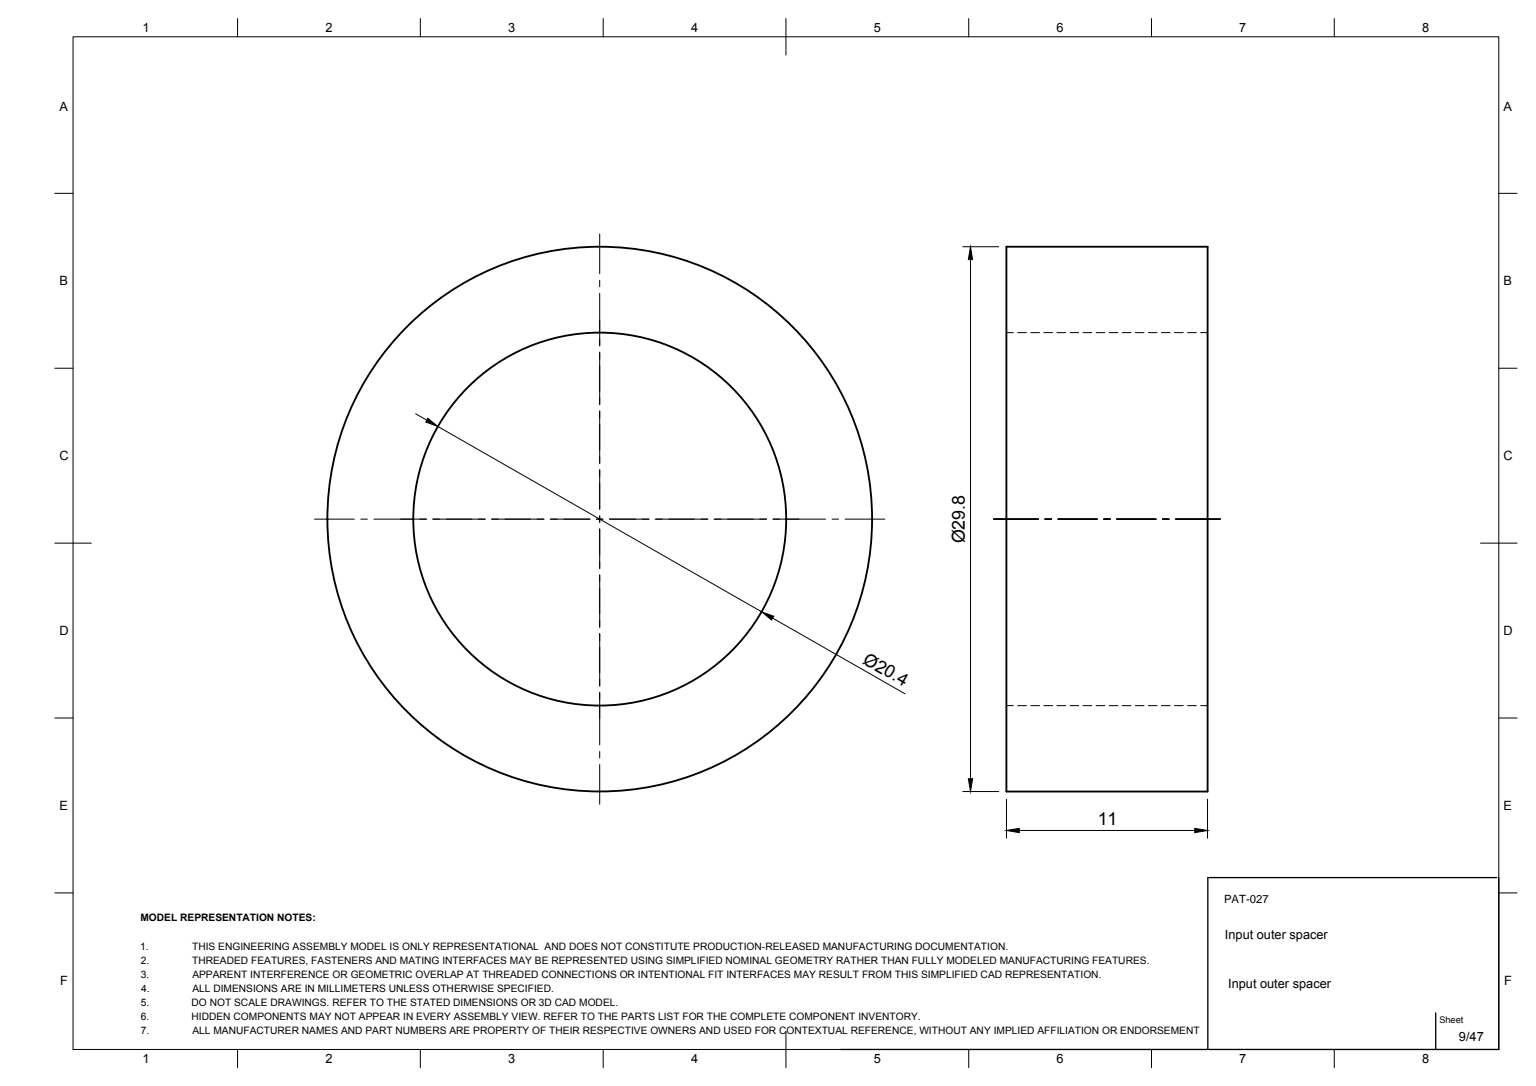
ISO-10303-21;
HEADER;
/* Generated by software containing ST-Developer
 * from STEP Tools, Inc. (www.steptools.com) 
 */

FILE_DESCRIPTION(
/* description */ ('Crank-driven oscillating fan base (mechanism only)'),

/* implementation_level */ '2;1');

FILE_NAME(
/* name */ 'Input outer spacer.step',
/* time_stamp */ '2026-10-28T03:25:00-07:00',
/* author */ (''),
/* organization */ (''),
/* preprocessor_version */ 'ST-DEVELOPER v20.2',
/* originating_system */ 'Autodesk Translation Framework v15.17.0.0',
/* authorisation */ '');

FILE_SCHEMA (('AUTOMOTIVE_DESIGN { 1 0 10303 214 3 1 1 }'));
ENDSEC;

DATA;
#10=MECHANICAL_DESIGN_GEOMETRIC_PRESENTATION_REPRESENTATION('',(#441),#11916);
#361=SHAPE_REPRESENTATION_RELATIONSHIP('SRR','None',#12085,#401);
#401=ADVANCED_BREP_SHAPE_REPRESENTATION('',(#489),#11876);
#441=STYLED_ITEM('',(#12368),#489);
#489=MANIFOLD_SOLID_BREP('Body1',#6071);
#564=FACE_BOUND('',#1353,.T.);
#565=FACE_BOUND('',#1355,.T.);
#722=PLANE('',#6683);
#723=PLANE('',#6684);
#941=FACE_OUTER_BOUND('',#1350,.T.);
#942=FACE_OUTER_BOUND('',#1351,.T.);
#943=FACE_OUTER_BOUND('',#1352,.T.);
#944=FACE_OUTER_BOUND('',#1354,.T.);
#1350=EDGE_LOOP('',(#4318,#4319,#4320,#4321));
#1351=EDGE_LOOP('',(#4322,#4323,#4324,#4325));
#1352=EDGE_LOOP('',(#4326));
#1353=EDGE_LOOP('',(#4327));
#1354=EDGE_LOOP('',(#4328));
#1355=EDGE_LOOP('',(#4329));
#1863=LINE('',#9791,#2196);
#1864=LINE('',#9797,#2197);
#2196=VECTOR('',#7716,1.02);
#2197=VECTOR('',#7723,1.49);
#2520=CIRCLE('',#6678,1.02);
#2521=CIRCLE('',#6679,1.02);
#2522=CIRCLE('',#6681,1.49);
#2523=CIRCLE('',#6682,1.49);
#2913=VERTEX_POINT('',#9788);
#2914=VERTEX_POINT('',#9790);
#2915=VERTEX_POINT('',#9794);
#2916=VERTEX_POINT('',#9796);
#3454=EDGE_CURVE('',#2913,#2913,#2520,.T.);
#3455=EDGE_CURVE('',#2913,#2914,#1863,.T.);
#3456=EDGE_CURVE('',#2914,#2914,#2521,.T.);
#3457=EDGE_CURVE('',#2915,#2915,#2522,.T.);
#3458=EDGE_CURVE('',#2915,#2916,#1864,.T.);
#3459=EDGE_CURVE('',#2916,#2916,#2523,.T.);
#4318=ORIENTED_EDGE('',*,*,#3454,.F.);
#4319=ORIENTED_EDGE('',*,*,#3455,.T.);
#4320=ORIENTED_EDGE('',*,*,#3456,.T.);
#4321=ORIENTED_EDGE('',*,*,#3455,.F.);
#4322=ORIENTED_EDGE('',*,*,#3457,.F.);
#4323=ORIENTED_EDGE('',*,*,#3458,.T.);
#4324=ORIENTED_EDGE('',*,*,#3459,.T.);
#4325=ORIENTED_EDGE('',*,*,#3458,.F.);
#4326=ORIENTED_EDGE('',*,*,#3457,.T.);
#4327=ORIENTED_EDGE('',*,*,#3454,.T.);
#4328=ORIENTED_EDGE('',*,*,#3459,.F.);
#4329=ORIENTED_EDGE('',*,*,#3456,.F.);
#5571=CYLINDRICAL_SURFACE('',#6677,1.02);
#5572=CYLINDRICAL_SURFACE('',#6680,1.49);
#5747=ADVANCED_FACE('',(#941),#5571,.F.);
#5748=ADVANCED_FACE('',(#942),#5572,.T.);
#5749=ADVANCED_FACE('',(#943,#564),#722,.T.);
#5750=ADVANCED_FACE('',(#944,#565),#723,.F.);
#6071=CLOSED_SHELL('',(#5747,#5748,#5749,#5750));
#6676=AXIS2_PLACEMENT_3D('',#9786,#7710,#7711);
#6677=AXIS2_PLACEMENT_3D('',#9787,#7712,#7713);
#6678=AXIS2_PLACEMENT_3D('',#9789,#7714,#7715);
#6679=AXIS2_PLACEMENT_3D('',#9792,#7717,#7718);
#6680=AXIS2_PLACEMENT_3D('',#9793,#7719,#7720);
#6681=AXIS2_PLACEMENT_3D('',#9795,#7721,#7722);
#6682=AXIS2_PLACEMENT_3D('',#9798,#7724,#7725);
#6683=AXIS2_PLACEMENT_3D('',#9799,#7726,#7727);
#6684=AXIS2_PLACEMENT_3D('',#9800,#7728,#7729);
#7710=DIRECTION('axis',(0.,0.,1.));
#7711=DIRECTION('refdir',(1.,0.,0.));
#7712=DIRECTION('center_axis',(0.,0.,1.));
#7713=DIRECTION('ref_axis',(1.,0.,0.));
#7714=DIRECTION('center_axis',(0.,0.,-1.));
#7715=DIRECTION('ref_axis',(1.,0.,0.));
#7716=DIRECTION('',(0.,0.,-1.));
#7717=DIRECTION('center_axis',(0.,0.,-1.));
#7718=DIRECTION('ref_axis',(1.,0.,0.));
#7719=DIRECTION('center_axis',(0.,0.,1.));
#7720=DIRECTION('ref_axis',(1.,0.,0.));
#7721=DIRECTION('center_axis',(0.,0.,1.));
#7722=DIRECTION('ref_axis',(1.,0.,0.));
#7723=DIRECTION('',(0.,0.,-1.));
#7724=DIRECTION('center_axis',(0.,0.,1.));
#7725=DIRECTION('ref_axis',(1.,0.,0.));
#7726=DIRECTION('center_axis',(0.,0.,1.));
#7727=DIRECTION('ref_axis',(1.,0.,0.));
#7728=DIRECTION('center_axis',(0.,0.,1.));
#7729=DIRECTION('ref_axis',(1.,0.,0.));
#9786=CARTESIAN_POINT('',(0.,0.,0.));
#9787=CARTESIAN_POINT('Origin',(0.,0.,2.95));
#9788=CARTESIAN_POINT('',(-1.02,-1.2491397351303E-16,4.05));
#9789=CARTESIAN_POINT('Origin',(0.,0.,4.05));
#9790=CARTESIAN_POINT('',(-1.02,-1.2491397351303E-16,2.95));
#9791=CARTESIAN_POINT('',(-1.02,-1.2491397351303E-16,2.95));
#9792=CARTESIAN_POINT('Origin',(0.,0.,2.95));
#9793=CARTESIAN_POINT('Origin',(0.,0.,2.95));
#9794=CARTESIAN_POINT('',(-1.49,-1.82472373072956E-16,4.05));
#9795=CARTESIAN_POINT('Origin',(0.,0.,4.05));
#9796=CARTESIAN_POINT('',(-1.49,-1.82472373072956E-16,2.95));
#9797=CARTESIAN_POINT('',(-1.49,-1.82472373072956E-16,2.95));
#9798=CARTESIAN_POINT('Origin',(0.,0.,2.95));
#9799=CARTESIAN_POINT('Origin',(0.,0.,4.05));
#9800=CARTESIAN_POINT('Origin',(0.,0.,2.95));
#11829=UNCERTAINTY_MEASURE_WITH_UNIT(LENGTH_MEASURE(0.001),#11917,
'DISTANCE_ACCURACY_VALUE',
'Maximum model space distance between geometric entities at asserted c
onnectivities');
#11869=UNCERTAINTY_MEASURE_WITH_UNIT(LENGTH_MEASURE(0.001),#11917,
'DISTANCE_ACCURACY_VALUE',
'Maximum model space distance between geometric entities at asserted c
onnectivities');
#11876=(
GEOMETRIC_REPRESENTATION_CONTEXT(3)
GLOBAL_UNCERTAINTY_ASSIGNED_CONTEXT((#11829))
GLOBAL_UNIT_ASSIGNED_CONTEXT((#11917,#11919,#11920))
REPRESENTATION_CONTEXT('','3D')
);
#11916=(
GEOMETRIC_REPRESENTATION_CONTEXT(3)
GLOBAL_UNCERTAINTY_ASSIGNED_CONTEXT((#11869))
GLOBAL_UNIT_ASSIGNED_CONTEXT((#11917,#11919,#11920))
REPRESENTATION_CONTEXT('','3D')
);
#11917=(
LENGTH_UNIT()
NAMED_UNIT(*)
SI_UNIT(.CENTI.,.METRE.)
);
#11919=(
NAMED_UNIT(*)
PLANE_ANGLE_UNIT()
SI_UNIT($,.RADIAN.)
);
#11920=(
NAMED_UNIT(*)
SI_UNIT($,.STERADIAN.)
SOLID_ANGLE_UNIT()
);
#11927=SHAPE_DEFINITION_REPRESENTATION(#11973,#12085);
#11973=PRODUCT_DEFINITION_SHAPE('',$,#12132);
#12085=SHAPE_REPRESENTATION('',(#6676),#11876);
#12125=PRODUCT_DEFINITION_CONTEXT('part definition',#12265,'design');
#12132=PRODUCT_DEFINITION('Input outer spacer','Input outer spacer',#12178,
#12125);
#12178=PRODUCT_DEFINITION_FORMATION('',$,#12273);
#12265=APPLICATION_CONTEXT(
'Core Data for Automotive Mechanical Design Process');
#12266=PRODUCT_CONTEXT('part definition',#12265,'mechanical');
#12273=PRODUCT('Input outer spacer','Input outer spacer',
'Input outer spacer',(#12266));
#12362=COLOUR_RGB('Sky Blue',0.24,0.69,0.87);
#12363=FILL_AREA_STYLE_COLOUR('',#12362);
#12364=FILL_AREA_STYLE('',(#12363));
#12365=SURFACE_STYLE_FILL_AREA(#12364);
#12366=SURFACE_SIDE_STYLE('',(#12365));
#12367=SURFACE_STYLE_USAGE(.BOTH.,#12366);
#12368=PRESENTATION_STYLE_ASSIGNMENT((#12367));
ENDSEC;
END-ISO-10303-21;
